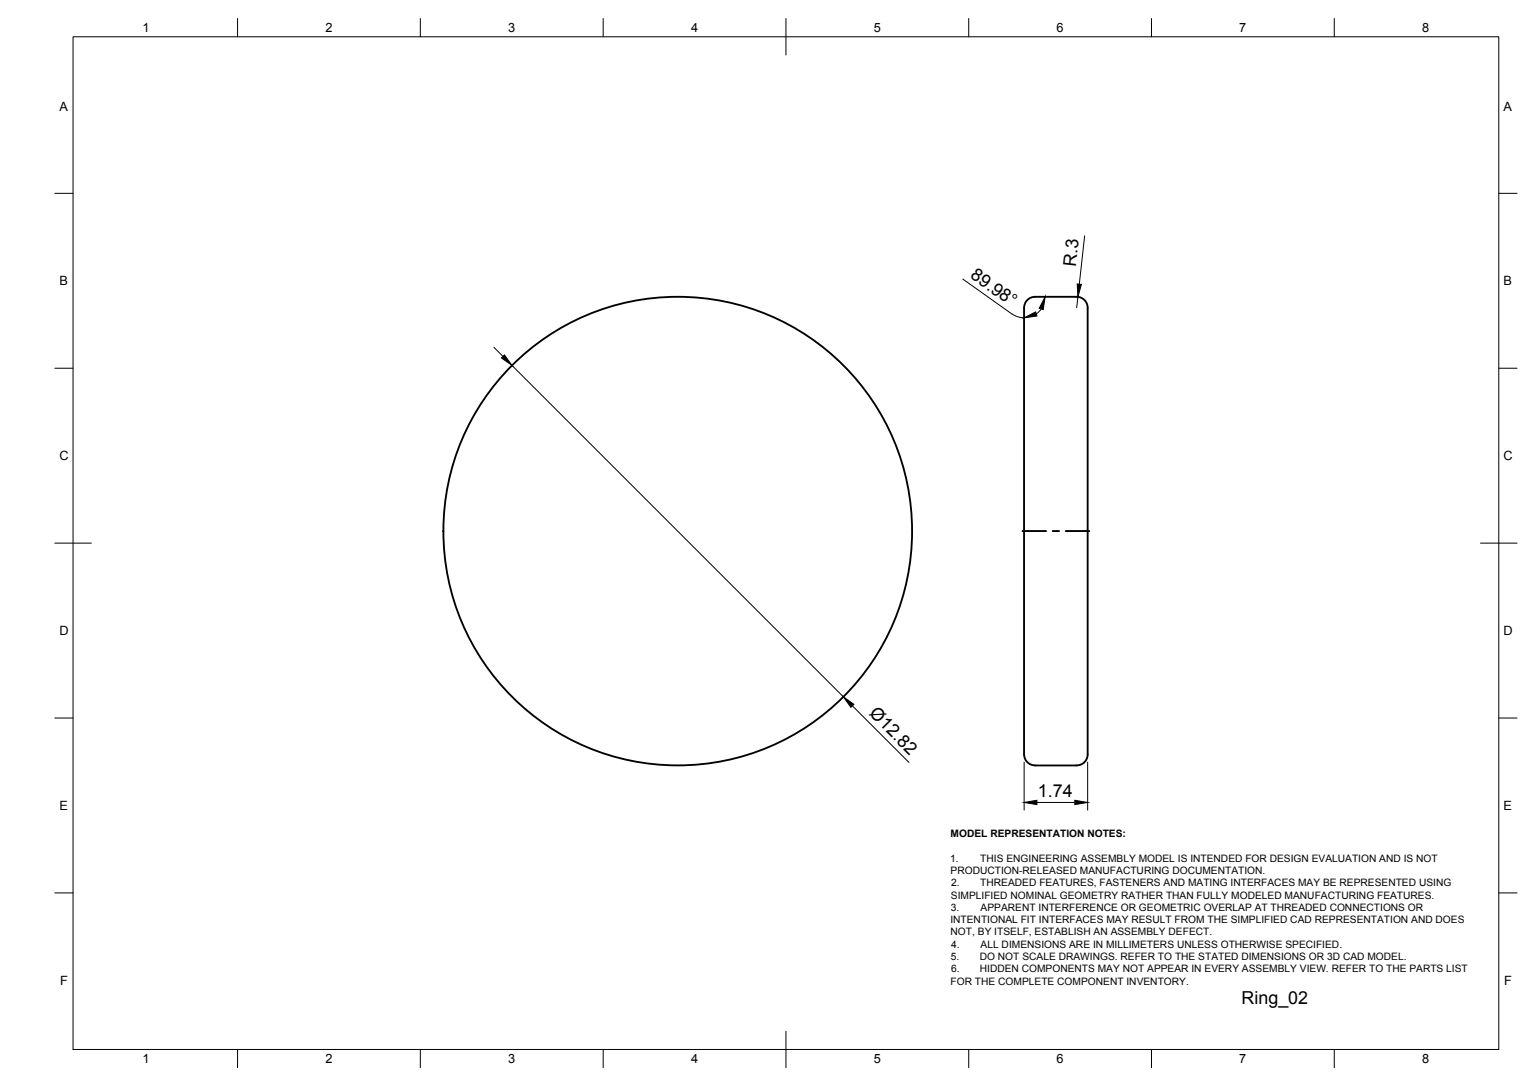
ISO-10303-21;
HEADER;
/* Generated by software containing ST-Developer
 * from STEP Tools, Inc. (www.steptools.com) 
 */

FILE_DESCRIPTION(
/* description */ (''),
/* implementation_level */ '2;1');

FILE_NAME(
/* name */ 'Ring_02.step',
/* time_stamp */ '2026-10-06T13:05:37-07:00',
/* author */ (''),
/* organization */ (''),
/* preprocessor_version */ 'ST-DEVELOPER v20.2',
/* originating_system */ 'Autodesk Translation Framework v15.15.0.0',
/* authorisation */ '');

FILE_SCHEMA (('AUTOMOTIVE_DESIGN { 1 0 10303 214 3 1 1 }'));
ENDSEC;

DATA;
#10=MECHANICAL_DESIGN_GEOMETRIC_PRESENTATION_REPRESENTATION('',(#140),#28055);
#110=TOROIDAL_SURFACE('',#3991,6.10923539706593,0.3);
#111=TOROIDAL_SURFACE('',#3998,6.1088989677085,0.3);
#120=SHAPE_REPRESENTATION_RELATIONSHIP('SRR','None',#28097,#130);
#130=ADVANCED_BREP_SHAPE_REPRESENTATION('',(#150),#28049);
#140=STYLED_ITEM('',(#28153),#150);
#150=MANIFOLD_SOLID_BREP('Body1',#3681);
#169=CONICAL_SURFACE('',#3995,6.40906719549494,0.00029560929023293);
#233=PLANE('',#3997);
#234=PLANE('',#4001);
#343=CIRCLE('',#3992,6.10923539706593);
#344=CIRCLE('',#3993,0.3);
#345=CIRCLE('',#3994,6.4092353839582);
#346=CIRCLE('',#3996,6.40889895460077);
#347=CIRCLE('',#3999,0.3);
#348=CIRCLE('',#4000,6.1088989677085);
#485=FACE_OUTER_BOUND('',#714,.T.);
#486=FACE_OUTER_BOUND('',#715,.T.);
#487=FACE_OUTER_BOUND('',#716,.T.);
#488=FACE_OUTER_BOUND('',#717,.T.);
#489=FACE_OUTER_BOUND('',#718,.T.);
#714=EDGE_LOOP('',(#2900,#2901,#2902,#2903));
#715=EDGE_LOOP('',(#2904,#2905,#2906,#2907));
#716=EDGE_LOOP('',(#2908));
#717=EDGE_LOOP('',(#2909,#2910,#2911,#2912));
#718=EDGE_LOOP('',(#2913));
#892=LINE('',#22128,#1050);
#1050=VECTOR('',#4577,6.40906719549494);
#1606=VERTEX_POINT('',#22121);
#1607=VERTEX_POINT('',#22123);
#1608=VERTEX_POINT('',#22127);
#1609=VERTEX_POINT('',#22132);
#2063=EDGE_CURVE('',#1606,#1606,#343,.T.);
#2064=EDGE_CURVE('',#1606,#1607,#344,.T.);
#2065=EDGE_CURVE('',#1607,#1607,#345,.T.);
#2066=EDGE_CURVE('',#1607,#1608,#892,.T.);
#2067=EDGE_CURVE('',#1608,#1608,#346,.T.);
#2068=EDGE_CURVE('',#1608,#1609,#347,.T.);
#2069=EDGE_CURVE('',#1609,#1609,#348,.T.);
#2900=ORIENTED_EDGE('',*,*,#2063,.T.);
#2901=ORIENTED_EDGE('',*,*,#2064,.T.);
#2902=ORIENTED_EDGE('',*,*,#2065,.T.);
#2903=ORIENTED_EDGE('',*,*,#2064,.F.);
#2904=ORIENTED_EDGE('',*,*,#2065,.F.);
#2905=ORIENTED_EDGE('',*,*,#2066,.T.);
#2906=ORIENTED_EDGE('',*,*,#2067,.F.);
#2907=ORIENTED_EDGE('',*,*,#2066,.F.);
#2908=ORIENTED_EDGE('',*,*,#2063,.F.);
#2909=ORIENTED_EDGE('',*,*,#2067,.T.);
#2910=ORIENTED_EDGE('',*,*,#2068,.T.);
#2911=ORIENTED_EDGE('',*,*,#2069,.T.);
#2912=ORIENTED_EDGE('',*,*,#2068,.F.);
#2913=ORIENTED_EDGE('',*,*,#2069,.F.);
#3577=ADVANCED_FACE('',(#485),#110,.T.);
#3578=ADVANCED_FACE('',(#486),#169,.T.);
#3579=ADVANCED_FACE('',(#487),#233,.T.);
#3580=ADVANCED_FACE('',(#488),#111,.T.);
#3581=ADVANCED_FACE('',(#489),#234,.T.);
#3681=CLOSED_SHELL('',(#3577,#3578,#3579,#3580,#3581));
#3990=AXIS2_PLACEMENT_3D('',#22119,#4565,#4566);
#3991=AXIS2_PLACEMENT_3D('',#22120,#4567,#4568);
#3992=AXIS2_PLACEMENT_3D('',#22122,#4569,#4570);
#3993=AXIS2_PLACEMENT_3D('',#22124,#4571,#4572);
#3994=AXIS2_PLACEMENT_3D('',#22125,#4573,#4574);
#3995=AXIS2_PLACEMENT_3D('',#22126,#4575,#4576);
#3996=AXIS2_PLACEMENT_3D('',#22129,#4578,#4579);
#3997=AXIS2_PLACEMENT_3D('',#22130,#4580,#4581);
#3998=AXIS2_PLACEMENT_3D('',#22131,#4582,#4583);
#3999=AXIS2_PLACEMENT_3D('',#22133,#4584,#4585);
#4000=AXIS2_PLACEMENT_3D('',#22134,#4586,#4587);
#4001=AXIS2_PLACEMENT_3D('',#22135,#4588,#4589);
#4565=DIRECTION('axis',(0.,0.,1.));
#4566=DIRECTION('refdir',(1.,0.,0.));
#4567=DIRECTION('center_axis',(1.,0.,0.));
#4568=DIRECTION('ref_axis',(0.,0.,-1.));
#4569=DIRECTION('center_axis',(-1.,0.,0.));
#4570=DIRECTION('ref_axis',(0.,1.22464679914735E-16,1.));
#4571=DIRECTION('center_axis',(0.,-1.,-1.22464679914735E-16));
#4572=DIRECTION('ref_axis',(0.,-1.22464679914735E-16,1.));
#4573=DIRECTION('center_axis',(1.,0.,0.));
#4574=DIRECTION('ref_axis',(0.,0.,1.));
#4575=DIRECTION('center_axis',(1.,0.,0.));
#4576=DIRECTION('ref_axis',(0.,0.,-1.));
#4577=DIRECTION('',(-0.999999956307574,3.62016965809512E-20,-0.000295609285927634));
#4578=DIRECTION('center_axis',(-1.,0.,0.));
#4579=DIRECTION('ref_axis',(0.,0.,1.));
#4580=DIRECTION('center_axis',(1.,0.,0.));
#4581=DIRECTION('ref_axis',(0.,0.,-1.));
#4582=DIRECTION('center_axis',(1.,0.,0.));
#4583=DIRECTION('ref_axis',(0.,0.,-1.));
#4584=DIRECTION('center_axis',(0.,-1.,-1.22464679914735E-16));
#4585=DIRECTION('ref_axis',(0.,-1.22464679914735E-16,1.));
#4586=DIRECTION('center_axis',(1.,0.,0.));
#4587=DIRECTION('ref_axis',(0.,1.22464679914735E-16,1.));
#4588=DIRECTION('center_axis',(-1.,0.,0.));
#4589=DIRECTION('ref_axis',(0.,0.,1.));
#22119=CARTESIAN_POINT('',(0.,0.,0.));
#22120=CARTESIAN_POINT('Origin',(30.1110679337117,0.,0.));
#22121=CARTESIAN_POINT('',(30.4110679337117,-7.4816555742545E-16,6.10923539706593));
#22122=CARTESIAN_POINT('Origin',(30.4110679337117,0.,0.));
#22123=CARTESIAN_POINT('',(30.1109792509259,-7.84904959794637E-16,6.4092353839582));
#22124=CARTESIAN_POINT('Origin',(30.1110679337117,-7.4816555742545E-16,
6.10923539706593));
#22125=CARTESIAN_POINT('Origin',(30.1109792509259,-7.84904959794637E-16,
0.));
#22126=CARTESIAN_POINT('Origin',(29.5420239984498,0.,0.));
#22127=CARTESIAN_POINT('',(28.9728913804021,-7.84863759081066E-16,6.40889895460077));
#22128=CARTESIAN_POINT('',(29.5420239984498,-7.84884362648318E-16,6.40906719549494));
#22129=CARTESIAN_POINT('Origin',(28.9728913804021,-7.84863759081066E-16,
0.));
#22130=CARTESIAN_POINT('Origin',(30.4110679337117,0.,0.));
#22131=CARTESIAN_POINT('Origin',(28.9729800631879,0.,0.));
#22132=CARTESIAN_POINT('',(28.6729800631879,-7.48124356711879E-16,6.1088989677085));
#22133=CARTESIAN_POINT('Origin',(28.9729800631879,-7.48124356711878E-16,
6.1088989677085));
#22134=CARTESIAN_POINT('Origin',(28.6729800631879,0.,0.));
#22135=CARTESIAN_POINT('Origin',(28.6729800631879,0.,-6.40881029802658));
#28037=UNCERTAINTY_MEASURE_WITH_UNIT(LENGTH_MEASURE(0.01),#28056,
'DISTANCE_ACCURACY_VALUE',
'Maximum model space distance between geometric entities at asserted c
onnectivities');
#28043=UNCERTAINTY_MEASURE_WITH_UNIT(LENGTH_MEASURE(0.01),#28056,
'DISTANCE_ACCURACY_VALUE',
'Maximum model space distance between geometric entities at asserted c
onnectivities');
#28049=(
GEOMETRIC_REPRESENTATION_CONTEXT(3)
GLOBAL_UNCERTAINTY_ASSIGNED_CONTEXT((#28037))
GLOBAL_UNIT_ASSIGNED_CONTEXT((#28056,#28058,#28059))
REPRESENTATION_CONTEXT('','3D')
);
#28055=(
GEOMETRIC_REPRESENTATION_CONTEXT(3)
GLOBAL_UNCERTAINTY_ASSIGNED_CONTEXT((#28043))
GLOBAL_UNIT_ASSIGNED_CONTEXT((#28056,#28058,#28059))
REPRESENTATION_CONTEXT('','3D')
);
#28056=(
LENGTH_UNIT()
NAMED_UNIT(*)
SI_UNIT(.MILLI.,.METRE.)
);
#28058=(
NAMED_UNIT(*)
PLANE_ANGLE_UNIT()
SI_UNIT($,.RADIAN.)
);
#28059=(
NAMED_UNIT(*)
SI_UNIT($,.STERADIAN.)
SOLID_ANGLE_UNIT()
);
#28065=SHAPE_DEFINITION_REPRESENTATION(#28076,#28097);
#28076=PRODUCT_DEFINITION_SHAPE('',$,#28109);
#28097=SHAPE_REPRESENTATION('',(#3990),#28049);
#28103=PRODUCT_DEFINITION_CONTEXT('part definition',#28138,'design');
#28109=PRODUCT_DEFINITION('Ring_02','Ring_02',#28120,#28103);
#28120=PRODUCT_DEFINITION_FORMATION('',$,#28145);
#28138=APPLICATION_CONTEXT(
'Core Data for Automotive Mechanical Design Process');
#28139=PRODUCT_CONTEXT('part definition',#28138,'mechanical');
#28145=PRODUCT('Ring_02','Ring_02',$,(#28139));
#28153=PRESENTATION_STYLE_ASSIGNMENT((#28156));
#28156=SURFACE_STYLE_USAGE(.BOTH.,#28159);
#28159=SURFACE_SIDE_STYLE('',(#28162));
#28162=SURFACE_STYLE_FILL_AREA(#28165);
#28165=FILL_AREA_STYLE('Opaque(39,39,39)',(#28168));
#28168=FILL_AREA_STYLE_COLOUR('Opaque(39,39,39)',#28171);
#28171=COLOUR_RGB('Opaque(39,39,39)', 0.08235294, 0.09019608, 0.10196078);
ENDSEC;
END-ISO-10303-21;
